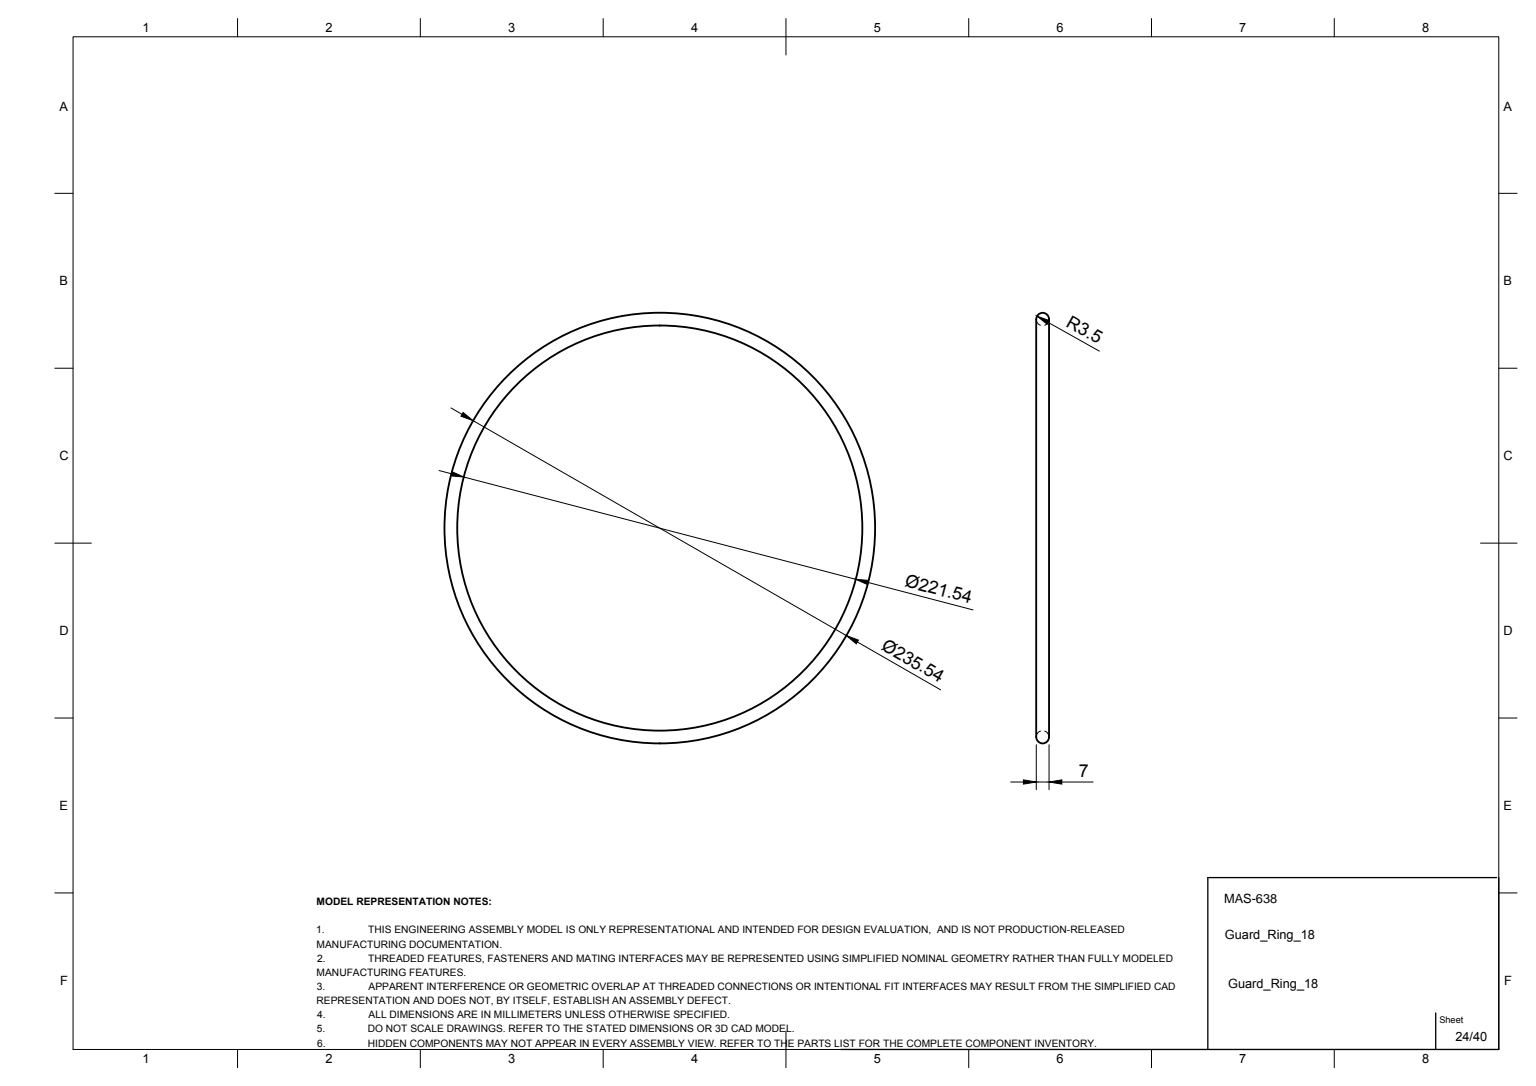
ISO-10303-21;
HEADER;
FILE_DESCRIPTION((''),'2;1');
FILE_NAME('Guard_Ring_18.step','2026-10-09T12:00:21-07:00',(''),(''),'','','');
FILE_SCHEMA (('AUTOMOTIVE_DESIGN { 1 0 10303 214 3 1 1 }'));
ENDSEC;
DATA;
#10=MECHANICAL_DESIGN_GEOMETRIC_PRESENTATION_REPRESENTATION('',(#423),#10334);
#351=SHAPE_REPRESENTATION_RELATIONSHIP('SRR','None',#10467,#383) ;
#383=ADVANCED_BREP_SHAPE_REPRESENTATION('',(#455),#10319) ;
#423=STYLED_ITEM('',(#10631),#455) ;
#455=MANIFOLD_SOLID_BREP('Body1',#3577) ;
#876=FACE_OUTER_BOUND('',#1076,.T.) ;
#1076=EDGE_LOOP('',(#2417,#2418,#2419,#2420)) ;
#1310=CIRCLE('',#4043,0.349999999999999) ;
#1311=CIRCLE('',#4044,11.0768144613668) ;
#1530=VERTEX_POINT('',#5738) ;
#1865=EDGE_CURVE('',#1530,#1530,#1310,.T.) ;
#1866=EDGE_CURVE('',#1530,#1530,#1311,.T.) ;
#2417=ORIENTED_EDGE('',*,*,#1865,.F.) ;
#2418=ORIENTED_EDGE('',*,*,#1866,.T.) ;
#2419=ORIENTED_EDGE('',*,*,#1865,.T.) ;
#2420=ORIENTED_EDGE('',*,*,#1866,.F.) ;
#3322=TOROIDAL_SURFACE('',#4042,11.4268144613668,0.349999999999999) ;
#3384=ADVANCED_FACE('',(#876),#3322,.T.) ;
#3577=CLOSED_SHELL('',(#3384)) ;
#4041=AXIS2_PLACEMENT_3D('',#5736,#4643,#4644) ;
#4042=AXIS2_PLACEMENT_3D('',#5737,#4645,#4646) ;
#4043=AXIS2_PLACEMENT_3D('',#5739,#4647,#4648) ;
#4044=AXIS2_PLACEMENT_3D('',#5740,#4649,#4650) ;
#4643=DIRECTION('axis',(0.,0.,1.)) ;
#4644=DIRECTION('refdir',(1.,0.,0.)) ;
#4645=DIRECTION('center_axis',(-6.42891162084177E-17,-1.,-1.01883556321148E-16)) ;
#4646=DIRECTION('ref_axis',(1.,0.,0.)) ;
#4647=DIRECTION('center_axis',(0.,1.01883556321148E-16,-1.)) ;
#4648=DIRECTION('ref_axis',(-1.,0.,0.)) ;
#4649=DIRECTION('center_axis',(6.42891162084177E-17,1.,1.01883556321148E-16)) ;
#4650=DIRECTION('ref_axis',(1.,-6.42891162084177E-17,-6.55000379205715E-33)) ;
#5736=CARTESIAN_POINT('',(0.,0.,0.)) ;
#5737=CARTESIAN_POINT('Origin',(23.47768801576,65.2831179463143,68.2224337400009)) ;
#5738=CARTESIAN_POINT('',(12.4008735543932,65.2831179463143,68.2224337400009)) ;
#5739=CARTESIAN_POINT('Origin',(12.0508735543932,65.2831179463143,68.2224337400009)) ;
#5740=CARTESIAN_POINT('Origin',(23.47768801576,65.2831179463143,68.2224337400009)) ;
#10282=UNCERTAINTY_MEASURE_WITH_UNIT(LENGTH_MEASURE(0.001),#10335,
'DISTANCE_ACCURACY_VALUE',
'Maximum model space distance between geometric entities at asserted c
onnectivities') ;
#10297=UNCERTAINTY_MEASURE_WITH_UNIT(LENGTH_MEASURE(0.001),#10335,
'DISTANCE_ACCURACY_VALUE',
'Maximum model space distance between geometric entities at asserted c
onnectivities') ;
#10319=(
GEOMETRIC_REPRESENTATION_CONTEXT(3)
GLOBAL_UNCERTAINTY_ASSIGNED_CONTEXT((#10282))
GLOBAL_UNIT_ASSIGNED_CONTEXT((#10335,#10337,#10338))
REPRESENTATION_CONTEXT('','3D')
) ;
#10334=(
GEOMETRIC_REPRESENTATION_CONTEXT(3)
GLOBAL_UNCERTAINTY_ASSIGNED_CONTEXT((#10297))
GLOBAL_UNIT_ASSIGNED_CONTEXT((#10335,#10337,#10338))
REPRESENTATION_CONTEXT('','3D')
) ;
#10335=(
LENGTH_UNIT()
NAMED_UNIT(*)
SI_UNIT(.CENTI.,.METRE.)
) ;
#10337=(
NAMED_UNIT(*)
PLANE_ANGLE_UNIT()
SI_UNIT($,.RADIAN.)
) ;
#10338=(
NAMED_UNIT(*)
SI_UNIT($,.STERADIAN.)
SOLID_ANGLE_UNIT()
) ;
#10360=SHAPE_DEFINITION_REPRESENTATION(#10396,#10467) ;
#10396=PRODUCT_DEFINITION_SHAPE('',$,#10504) ;
#10467=SHAPE_REPRESENTATION('',(#4041),#10319) ;
#10482=PRODUCT_DEFINITION_CONTEXT('part definition',#10592,'design') ;
#10504=PRODUCT_DEFINITION('Guard_Ring_18','Guard_Ring_18',#10540,#10482) ;
#10540=PRODUCT_DEFINITION_FORMATION('',$,#10615) ;
#10592=APPLICATION_CONTEXT(
'Core Data for Automotive Mechanical Design Process') ;
#10593=PRODUCT_CONTEXT('part definition',#10592,'mechanical') ;
#10615=PRODUCT('Guard_Ring_18','Guard_Ring_18',$,(#10593)) ;
#10631=PRESENTATION_STYLE_ASSIGNMENT((#10635)) ;
#10635=SURFACE_STYLE_USAGE(.BOTH.,#10639) ;
#10639=SURFACE_SIDE_STYLE('',(#10643)) ;
#10643=SURFACE_STYLE_FILL_AREA(#10647) ;
#10647=FILL_AREA_STYLE('Opaque(25,25,25)',(#10651)) ;
#10651=FILL_AREA_STYLE_COLOUR('Opaque(25,25,25)',#10655) ;
#10655=COLOUR_RGB('Opaque(25,25,25)', 0.09019608, 0.27058824, 0.51372549) ;
ENDSEC;
END-ISO-10303-21;
